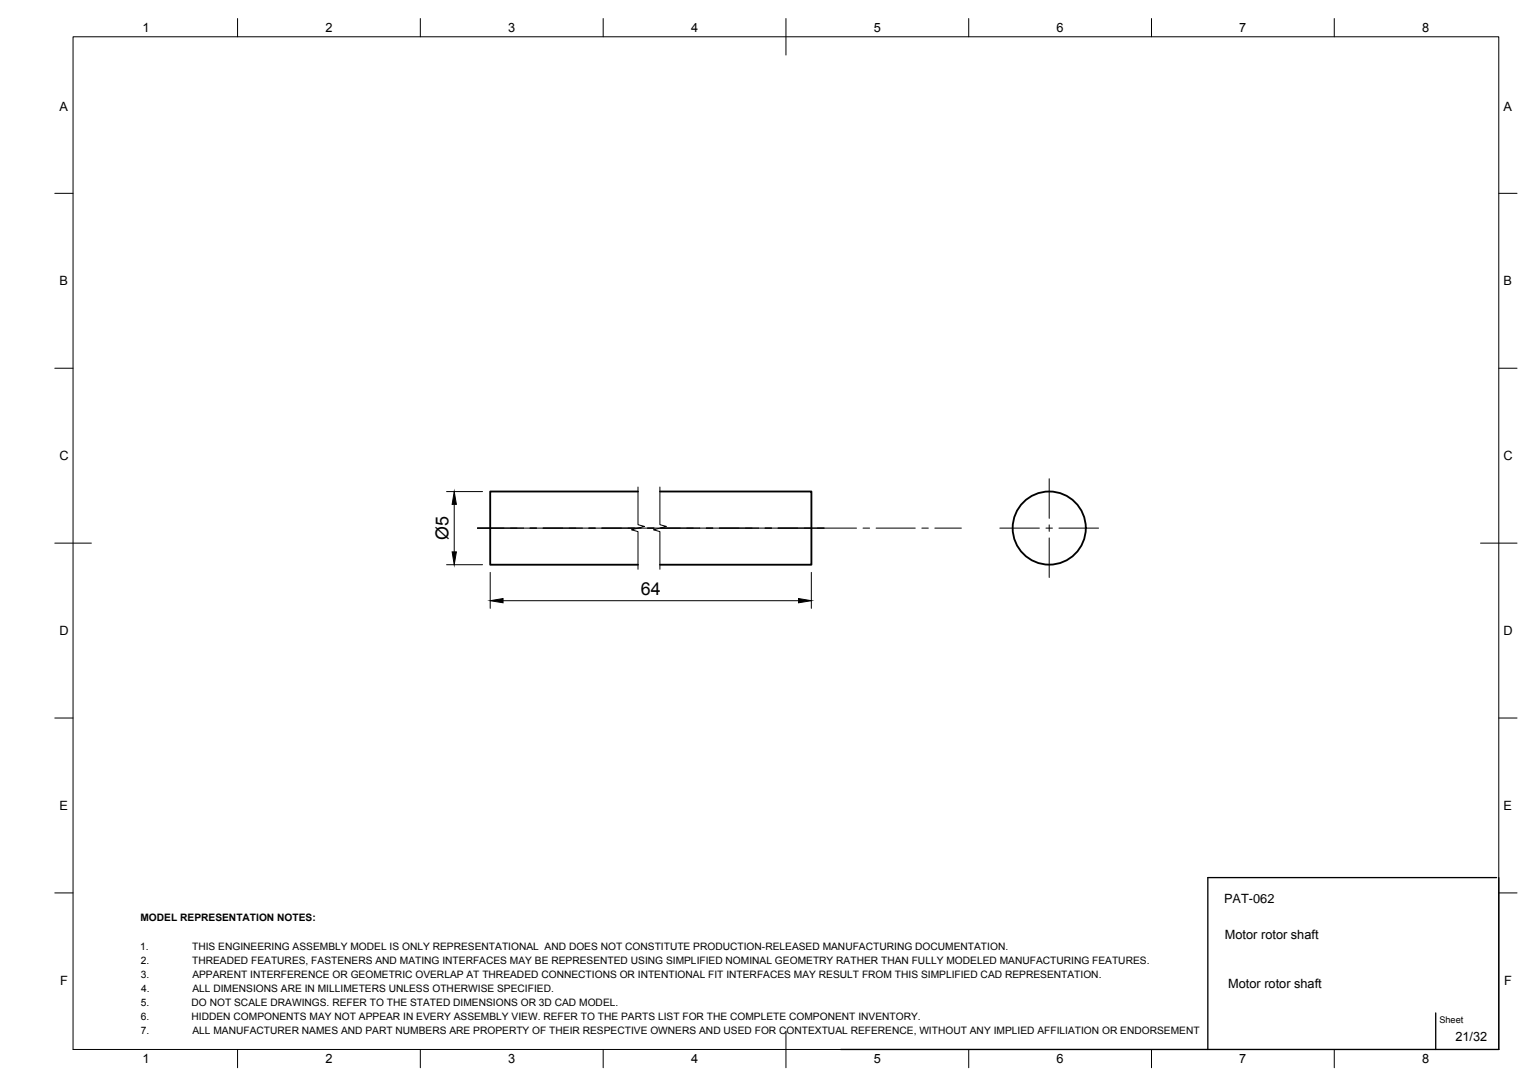
ISO-10303-21;
HEADER;
/* Generated by software containing ST-Developer
 * from STEP Tools, Inc. (www.steptools.com) 
 */

FILE_DESCRIPTION(
/* description */ ('Jaw-coupled motor to shaft test stand'),
/* implementation_level */ '2;1');

FILE_NAME(
/* name */ 'Motor rotor shaft.step',
/* time_stamp */ '2026-10-27T10:46:06-07:00',
/* author */ (''),
/* organization */ (''),
/* preprocessor_version */ 'ST-DEVELOPER v20.2',
/* originating_system */ 'Autodesk Translation Framework v15.17.0.0',
/* authorisation */ '');

FILE_SCHEMA (('AUTOMOTIVE_DESIGN { 1 0 10303 214 3 1 1 }'));
ENDSEC;

DATA;
#10=MECHANICAL_DESIGN_GEOMETRIC_PRESENTATION_REPRESENTATION('',(#360),#19361);
#295=SHAPE_REPRESENTATION_RELATIONSHIP('SRR','None',#19511,#327);
#327=ADVANCED_BREP_SHAPE_REPRESENTATION('',(#391),#19347);
#360=STYLED_ITEM('',(#19746),#391);
#391=MANIFOLD_SOLID_BREP('Body1',#11006);
#660=PLANE('',#11764);
#661=PLANE('',#11765);
#1233=FACE_OUTER_BOUND('',#1935,.T.);
#1234=FACE_OUTER_BOUND('',#1936,.T.);
#1235=FACE_OUTER_BOUND('',#1937,.T.);
#1935=EDGE_LOOP('',(#8248,#8249,#8250,#8251));
#1936=EDGE_LOOP('',(#8252));
#1937=EDGE_LOOP('',(#8253));
#2676=LINE('',#16858,#3829);
#3829=VECTOR('',#13421,0.25);
#4807=CIRCLE('',#11762,0.25);
#4808=CIRCLE('',#11763,0.25);
#5249=VERTEX_POINT('',#16855);
#5250=VERTEX_POINT('',#16857);
#6335=EDGE_CURVE('',#5249,#5249,#4807,.T.);
#6336=EDGE_CURVE('',#5249,#5250,#2676,.T.);
#6337=EDGE_CURVE('',#5250,#5250,#4808,.T.);
#8248=ORIENTED_EDGE('',*,*,#6335,.F.);
#8249=ORIENTED_EDGE('',*,*,#6336,.T.);
#8250=ORIENTED_EDGE('',*,*,#6337,.T.);
#8251=ORIENTED_EDGE('',*,*,#6336,.F.);
#8252=ORIENTED_EDGE('',*,*,#6335,.T.);
#8253=ORIENTED_EDGE('',*,*,#6337,.F.);
#10329=CYLINDRICAL_SURFACE('',#11761,0.25);
#10575=ADVANCED_FACE('',(#1233),#10329,.T.);
#10576=ADVANCED_FACE('',(#1234),#660,.T.);
#10577=ADVANCED_FACE('',(#1235),#661,.F.);
#11006=CLOSED_SHELL('',(#10575,#10576,#10577));
#11760=AXIS2_PLACEMENT_3D('',#16853,#13415,#13416);
#11761=AXIS2_PLACEMENT_3D('',#16854,#13417,#13418);
#11762=AXIS2_PLACEMENT_3D('',#16856,#13419,#13420);
#11763=AXIS2_PLACEMENT_3D('',#16859,#13422,#13423);
#11764=AXIS2_PLACEMENT_3D('',#16860,#13424,#13425);
#11765=AXIS2_PLACEMENT_3D('',#16861,#13426,#13427);
#13415=DIRECTION('axis',(0.,0.,1.));
#13416=DIRECTION('refdir',(1.,0.,0.));
#13417=DIRECTION('center_axis',(0.,1.,0.));
#13418=DIRECTION('ref_axis',(1.,0.,0.));
#13419=DIRECTION('center_axis',(0.,1.,0.));
#13420=DIRECTION('ref_axis',(1.,0.,0.));
#13421=DIRECTION('',(0.,-1.,0.));
#13422=DIRECTION('center_axis',(0.,1.,0.));
#13423=DIRECTION('ref_axis',(1.,0.,0.));
#13424=DIRECTION('center_axis',(0.,1.,0.));
#13425=DIRECTION('ref_axis',(1.,0.,0.));
#13426=DIRECTION('center_axis',(0.,1.,0.));
#13427=DIRECTION('ref_axis',(1.,0.,0.));
#16853=CARTESIAN_POINT('',(0.,0.,0.));
#16854=CARTESIAN_POINT('Origin',(0.,-11.6,4.22));
#16855=CARTESIAN_POINT('',(-0.25,-5.2,4.22));
#16856=CARTESIAN_POINT('Origin',(0.,-5.2,4.22));
#16857=CARTESIAN_POINT('',(-0.25,-11.6,4.22));
#16858=CARTESIAN_POINT('',(-0.25,-11.6,4.22));
#16859=CARTESIAN_POINT('Origin',(0.,-11.6,4.22));
#16860=CARTESIAN_POINT('Origin',(0.,-5.2,4.22));
#16861=CARTESIAN_POINT('Origin',(0.,-11.6,4.22));
#19309=UNCERTAINTY_MEASURE_WITH_UNIT(LENGTH_MEASURE(0.001),#19362,
'DISTANCE_ACCURACY_VALUE',
'Maximum model space distance between geometric entities at asserted c
onnectivities');
#19323=UNCERTAINTY_MEASURE_WITH_UNIT(LENGTH_MEASURE(0.001),#19362,
'DISTANCE_ACCURACY_VALUE',
'Maximum model space distance between geometric entities at asserted c
onnectivities');
#19347=(
GEOMETRIC_REPRESENTATION_CONTEXT(3)
GLOBAL_UNCERTAINTY_ASSIGNED_CONTEXT((#19309))
GLOBAL_UNIT_ASSIGNED_CONTEXT((#19362,#19364,#19365))
REPRESENTATION_CONTEXT('','3D')
);
#19361=(
GEOMETRIC_REPRESENTATION_CONTEXT(3)
GLOBAL_UNCERTAINTY_ASSIGNED_CONTEXT((#19323))
GLOBAL_UNIT_ASSIGNED_CONTEXT((#19362,#19364,#19365))
REPRESENTATION_CONTEXT('','3D')
);
#19362=(
LENGTH_UNIT()
NAMED_UNIT(*)
SI_UNIT(.CENTI.,.METRE.)
);
#19364=(
NAMED_UNIT(*)
PLANE_ANGLE_UNIT()
SI_UNIT($,.RADIAN.)
);
#19365=(
NAMED_UNIT(*)
SI_UNIT($,.STERADIAN.)
SOLID_ANGLE_UNIT()
);
#19389=SHAPE_DEFINITION_REPRESENTATION(#19453,#19511);
#19453=PRODUCT_DEFINITION_SHAPE('',$,#19549);
#19511=SHAPE_REPRESENTATION('',(#11760),#19347);
#19525=PRODUCT_DEFINITION_CONTEXT('part definition',#19638,'design');
#19549=PRODUCT_DEFINITION('Motor rotor shaft','Motor rotor shaft',#19586,
#19525);
#19586=PRODUCT_DEFINITION_FORMATION('',$,#19663);
#19638=APPLICATION_CONTEXT(
'Core Data for Automotive Mechanical Design Process');
#19639=PRODUCT_CONTEXT('part definition',#19638,'mechanical');
#19663=PRODUCT('Motor rotor shaft','Motor rotor shaft',
'Motor rotor shaft',(#19639));
#19740=COLOUR_RGB('Grey',0.48,0.52,0.57);
#19741=FILL_AREA_STYLE_COLOUR('',#19740);
#19742=FILL_AREA_STYLE('',(#19741));
#19743=SURFACE_STYLE_FILL_AREA(#19742);
#19744=SURFACE_SIDE_STYLE('',(#19743));
#19745=SURFACE_STYLE_USAGE(.BOTH.,#19744);
#19746=PRESENTATION_STYLE_ASSIGNMENT((#19745));
ENDSEC;
END-ISO-10303-21;
